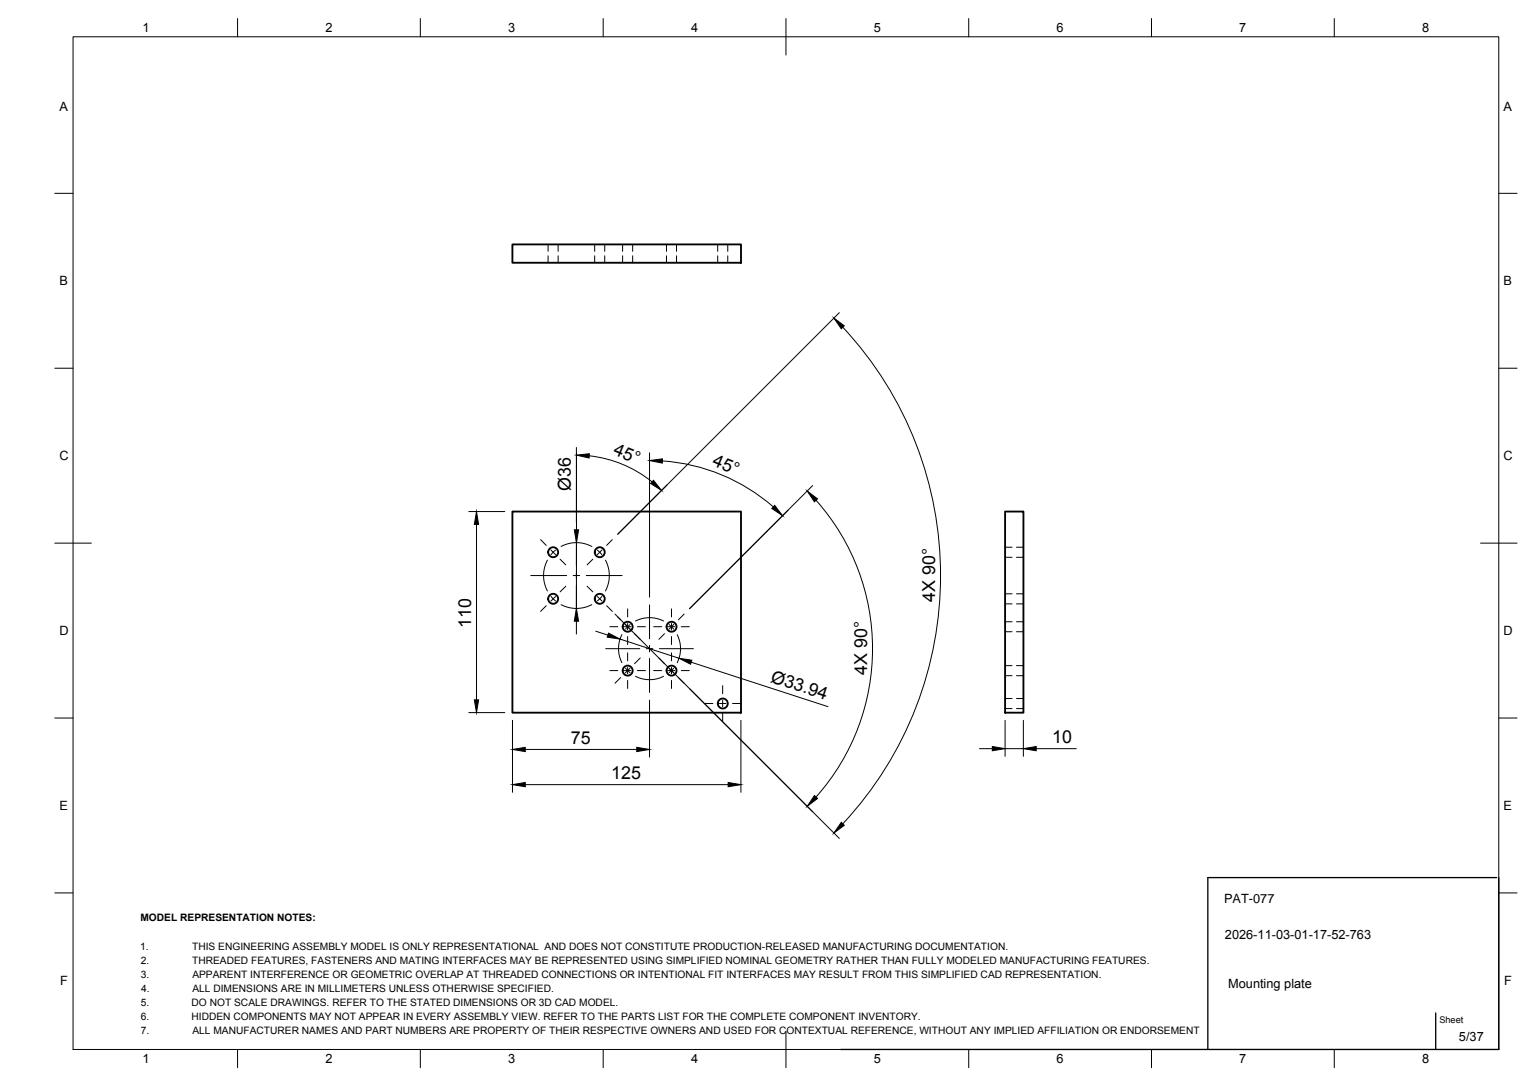
ISO-10303-21;
HEADER;
/* Generated by software containing ST-Developer
 * from STEP Tools, Inc. (www.steptools.com) 
 */

FILE_DESCRIPTION(
/* description */ ('Pallet stop with pneumatic fitting'),
/* implementation_level */ '2;1');

FILE_NAME(
/* name */ 'Mounting plate.step',
/* time_stamp */ '2026-10-27T10:51:41-07:00',
/* author */ (''),
/* organization */ (''),
/* preprocessor_version */ 'ST-DEVELOPER v20.2',
/* originating_system */ 'Autodesk Translation Framework v15.17.0.0',
/* authorisation */ '');

FILE_SCHEMA (('AUTOMOTIVE_DESIGN { 1 0 10303 214 3 1 1 }'));
ENDSEC;

DATA;
#10=MECHANICAL_DESIGN_GEOMETRIC_PRESENTATION_REPRESENTATION('',(#357),#10265);
#293=SHAPE_REPRESENTATION_RELATIONSHIP('SRR','None',#10406,#325);
#325=ADVANCED_BREP_SHAPE_REPRESENTATION('',(#389),#10230);
#357=STYLED_ITEM('',(#10641),#389);
#389=MANIFOLD_SOLID_BREP('Body1',#5045);
#419=FACE_BOUND('',#1064,.T.);
#420=FACE_BOUND('',#1065,.T.);
#421=FACE_BOUND('',#1066,.T.);
#422=FACE_BOUND('',#1067,.T.);
#423=FACE_BOUND('',#1068,.T.);
#424=FACE_BOUND('',#1069,.T.);
#425=FACE_BOUND('',#1070,.T.);
#426=FACE_BOUND('',#1071,.T.);
#427=FACE_BOUND('',#1072,.T.);
#428=FACE_BOUND('',#1074,.T.);
#429=FACE_BOUND('',#1075,.T.);
#430=FACE_BOUND('',#1076,.T.);
#431=FACE_BOUND('',#1077,.T.);
#432=FACE_BOUND('',#1078,.T.);
#433=FACE_BOUND('',#1079,.T.);
#434=FACE_BOUND('',#1080,.T.);
#435=FACE_BOUND('',#1081,.T.);
#436=FACE_BOUND('',#1082,.T.);
#545=PLANE('',#5462);
#546=PLANE('',#5463);
#547=PLANE('',#5464);
#548=PLANE('',#5465);
#549=PLANE('',#5466);
#550=PLANE('',#5467);
#736=FACE_OUTER_BOUND('',#1050,.T.);
#737=FACE_OUTER_BOUND('',#1051,.T.);
#738=FACE_OUTER_BOUND('',#1052,.T.);
#739=FACE_OUTER_BOUND('',#1053,.T.);
#740=FACE_OUTER_BOUND('',#1054,.T.);
#741=FACE_OUTER_BOUND('',#1055,.T.);
#742=FACE_OUTER_BOUND('',#1056,.T.);
#743=FACE_OUTER_BOUND('',#1057,.T.);
#744=FACE_OUTER_BOUND('',#1058,.T.);
#745=FACE_OUTER_BOUND('',#1059,.T.);
#746=FACE_OUTER_BOUND('',#1060,.T.);
#747=FACE_OUTER_BOUND('',#1061,.T.);
#748=FACE_OUTER_BOUND('',#1062,.T.);
#749=FACE_OUTER_BOUND('',#1063,.T.);
#750=FACE_OUTER_BOUND('',#1073,.T.);
#1050=EDGE_LOOP('',(#3410,#3411,#3412,#3413));
#1051=EDGE_LOOP('',(#3414,#3415,#3416,#3417));
#1052=EDGE_LOOP('',(#3418,#3419,#3420,#3421));
#1053=EDGE_LOOP('',(#3422,#3423,#3424,#3425));
#1054=EDGE_LOOP('',(#3426,#3427,#3428,#3429));
#1055=EDGE_LOOP('',(#3430,#3431,#3432,#3433));
#1056=EDGE_LOOP('',(#3434,#3435,#3436,#3437));
#1057=EDGE_LOOP('',(#3438,#3439,#3440,#3441));
#1058=EDGE_LOOP('',(#3442,#3443,#3444,#3445));
#1059=EDGE_LOOP('',(#3446,#3447,#3448,#3449));
#1060=EDGE_LOOP('',(#3450,#3451,#3452,#3453));
#1061=EDGE_LOOP('',(#3454,#3455,#3456,#3457));
#1062=EDGE_LOOP('',(#3458,#3459,#3460,#3461));
#1063=EDGE_LOOP('',(#3462,#3463,#3464,#3465));
#1064=EDGE_LOOP('',(#3466));
#1065=EDGE_LOOP('',(#3467));
#1066=EDGE_LOOP('',(#3468));
#1067=EDGE_LOOP('',(#3469));
#1068=EDGE_LOOP('',(#3470));
#1069=EDGE_LOOP('',(#3471));
#1070=EDGE_LOOP('',(#3472));
#1071=EDGE_LOOP('',(#3473));
#1072=EDGE_LOOP('',(#3474));
#1073=EDGE_LOOP('',(#3475,#3476,#3477,#3478));
#1074=EDGE_LOOP('',(#3479));
#1075=EDGE_LOOP('',(#3480));
#1076=EDGE_LOOP('',(#3481));
#1077=EDGE_LOOP('',(#3482));
#1078=EDGE_LOOP('',(#3483));
#1079=EDGE_LOOP('',(#3484));
#1080=EDGE_LOOP('',(#3485));
#1081=EDGE_LOOP('',(#3486));
#1082=EDGE_LOOP('',(#3487));
#1490=LINE('',#7745,#1825);
#1491=LINE('',#7751,#1826);
#1492=LINE('',#7757,#1827);
#1493=LINE('',#7763,#1828);
#1494=LINE('',#7769,#1829);
#1495=LINE('',#7775,#1830);
#1496=LINE('',#7781,#1831);
#1497=LINE('',#7787,#1832);
#1498=LINE('',#7793,#1833);
#1499=LINE('',#7798,#1834);
#1500=LINE('',#7800,#1835);
#1501=LINE('',#7802,#1836);
#1502=LINE('',#7803,#1837);
#1503=LINE('',#7806,#1838);
#1504=LINE('',#7808,#1839);
#1505=LINE('',#7809,#1840);
#1506=LINE('',#7812,#1841);
#1507=LINE('',#7814,#1842);
#1508=LINE('',#7815,#1843);
#1509=LINE('',#7817,#1844);
#1510=LINE('',#7818,#1845);
#1825=VECTOR('',#6099,0.275);
#1826=VECTOR('',#6106,0.275);
#1827=VECTOR('',#6113,0.275);
#1828=VECTOR('',#6120,0.275);
#1829=VECTOR('',#6127,0.275);
#1830=VECTOR('',#6134,0.275);
#1831=VECTOR('',#6141,0.275);
#1832=VECTOR('',#6148,0.275);
#1833=VECTOR('',#6155,0.275);
#1834=VECTOR('',#6160,1.);
#1835=VECTOR('',#6161,1.);
#1836=VECTOR('',#6162,1.);
#1837=VECTOR('',#6163,1.);
#1838=VECTOR('',#6166,1.);
#1839=VECTOR('',#6167,1.);
#1840=VECTOR('',#6168,1.);
#1841=VECTOR('',#6171,1.);
#1842=VECTOR('',#6172,1.);
#1843=VECTOR('',#6173,1.);
#1844=VECTOR('',#6176,1.);
#1845=VECTOR('',#6177,1.);
#2160=CIRCLE('',#5436,0.275);
#2161=CIRCLE('',#5437,0.275);
#2162=CIRCLE('',#5439,0.275);
#2163=CIRCLE('',#5440,0.275);
#2164=CIRCLE('',#5442,0.275);
#2165=CIRCLE('',#5443,0.275);
#2166=CIRCLE('',#5445,0.275);
#2167=CIRCLE('',#5446,0.275);
#2168=CIRCLE('',#5448,0.275);
#2169=CIRCLE('',#5449,0.275);
#2170=CIRCLE('',#5451,0.275);
#2171=CIRCLE('',#5452,0.275);
#2172=CIRCLE('',#5454,0.275);
#2173=CIRCLE('',#5455,0.275);
#2174=CIRCLE('',#5457,0.275);
#2175=CIRCLE('',#5458,0.275);
#2176=CIRCLE('',#5460,0.275);
#2177=CIRCLE('',#5461,0.275);
#2407=VERTEX_POINT('',#7742);
#2408=VERTEX_POINT('',#7744);
#2409=VERTEX_POINT('',#7748);
#2410=VERTEX_POINT('',#7750);
#2411=VERTEX_POINT('',#7754);
#2412=VERTEX_POINT('',#7756);
#2413=VERTEX_POINT('',#7760);
#2414=VERTEX_POINT('',#7762);
#2415=VERTEX_POINT('',#7766);
#2416=VERTEX_POINT('',#7768);
#2417=VERTEX_POINT('',#7772);
#2418=VERTEX_POINT('',#7774);
#2419=VERTEX_POINT('',#7778);
#2420=VERTEX_POINT('',#7780);
#2421=VERTEX_POINT('',#7784);
#2422=VERTEX_POINT('',#7786);
#2423=VERTEX_POINT('',#7790);
#2424=VERTEX_POINT('',#7792);
#2425=VERTEX_POINT('',#7796);
#2426=VERTEX_POINT('',#7797);
#2427=VERTEX_POINT('',#7799);
#2428=VERTEX_POINT('',#7801);
#2429=VERTEX_POINT('',#7805);
#2430=VERTEX_POINT('',#7807);
#2431=VERTEX_POINT('',#7811);
#2432=VERTEX_POINT('',#7813);
#2804=EDGE_CURVE('',#2407,#2407,#2160,.T.);
#2805=EDGE_CURVE('',#2407,#2408,#1490,.T.);
#2806=EDGE_CURVE('',#2408,#2408,#2161,.T.);
#2807=EDGE_CURVE('',#2409,#2409,#2162,.T.);
#2808=EDGE_CURVE('',#2409,#2410,#1491,.T.);
#2809=EDGE_CURVE('',#2410,#2410,#2163,.T.);
#2810=EDGE_CURVE('',#2411,#2411,#2164,.T.);
#2811=EDGE_CURVE('',#2411,#2412,#1492,.T.);
#2812=EDGE_CURVE('',#2412,#2412,#2165,.T.);
#2813=EDGE_CURVE('',#2413,#2413,#2166,.T.);
#2814=EDGE_CURVE('',#2413,#2414,#1493,.T.);
#2815=EDGE_CURVE('',#2414,#2414,#2167,.T.);
#2816=EDGE_CURVE('',#2415,#2415,#2168,.T.);
#2817=EDGE_CURVE('',#2415,#2416,#1494,.T.);
#2818=EDGE_CURVE('',#2416,#2416,#2169,.T.);
#2819=EDGE_CURVE('',#2417,#2417,#2170,.T.);
#2820=EDGE_CURVE('',#2417,#2418,#1495,.T.);
#2821=EDGE_CURVE('',#2418,#2418,#2171,.T.);
#2822=EDGE_CURVE('',#2419,#2419,#2172,.T.);
#2823=EDGE_CURVE('',#2419,#2420,#1496,.T.);
#2824=EDGE_CURVE('',#2420,#2420,#2173,.T.);
#2825=EDGE_CURVE('',#2421,#2421,#2174,.T.);
#2826=EDGE_CURVE('',#2421,#2422,#1497,.T.);
#2827=EDGE_CURVE('',#2422,#2422,#2175,.T.);
#2828=EDGE_CURVE('',#2423,#2423,#2176,.T.);
#2829=EDGE_CURVE('',#2423,#2424,#1498,.T.);
#2830=EDGE_CURVE('',#2424,#2424,#2177,.T.);
#2831=EDGE_CURVE('',#2425,#2426,#1499,.T.);
#2832=EDGE_CURVE('',#2426,#2427,#1500,.T.);
#2833=EDGE_CURVE('',#2428,#2427,#1501,.T.);
#2834=EDGE_CURVE('',#2425,#2428,#1502,.T.);
#2835=EDGE_CURVE('',#2429,#2425,#1503,.T.);
#2836=EDGE_CURVE('',#2430,#2428,#1504,.T.);
#2837=EDGE_CURVE('',#2429,#2430,#1505,.T.);
#2838=EDGE_CURVE('',#2431,#2429,#1506,.T.);
#2839=EDGE_CURVE('',#2432,#2430,#1507,.T.);
#2840=EDGE_CURVE('',#2431,#2432,#1508,.T.);
#2841=EDGE_CURVE('',#2426,#2431,#1509,.T.);
#2842=EDGE_CURVE('',#2427,#2432,#1510,.T.);
#3410=ORIENTED_EDGE('',*,*,#2804,.F.);
#3411=ORIENTED_EDGE('',*,*,#2805,.T.);
#3412=ORIENTED_EDGE('',*,*,#2806,.F.);
#3413=ORIENTED_EDGE('',*,*,#2805,.F.);
#3414=ORIENTED_EDGE('',*,*,#2807,.F.);
#3415=ORIENTED_EDGE('',*,*,#2808,.T.);
#3416=ORIENTED_EDGE('',*,*,#2809,.F.);
#3417=ORIENTED_EDGE('',*,*,#2808,.F.);
#3418=ORIENTED_EDGE('',*,*,#2810,.F.);
#3419=ORIENTED_EDGE('',*,*,#2811,.T.);
#3420=ORIENTED_EDGE('',*,*,#2812,.F.);
#3421=ORIENTED_EDGE('',*,*,#2811,.F.);
#3422=ORIENTED_EDGE('',*,*,#2813,.F.);
#3423=ORIENTED_EDGE('',*,*,#2814,.T.);
#3424=ORIENTED_EDGE('',*,*,#2815,.F.);
#3425=ORIENTED_EDGE('',*,*,#2814,.F.);
#3426=ORIENTED_EDGE('',*,*,#2816,.F.);
#3427=ORIENTED_EDGE('',*,*,#2817,.T.);
#3428=ORIENTED_EDGE('',*,*,#2818,.F.);
#3429=ORIENTED_EDGE('',*,*,#2817,.F.);
#3430=ORIENTED_EDGE('',*,*,#2819,.F.);
#3431=ORIENTED_EDGE('',*,*,#2820,.T.);
#3432=ORIENTED_EDGE('',*,*,#2821,.F.);
#3433=ORIENTED_EDGE('',*,*,#2820,.F.);
#3434=ORIENTED_EDGE('',*,*,#2822,.F.);
#3435=ORIENTED_EDGE('',*,*,#2823,.T.);
#3436=ORIENTED_EDGE('',*,*,#2824,.F.);
#3437=ORIENTED_EDGE('',*,*,#2823,.F.);
#3438=ORIENTED_EDGE('',*,*,#2825,.F.);
#3439=ORIENTED_EDGE('',*,*,#2826,.T.);
#3440=ORIENTED_EDGE('',*,*,#2827,.F.);
#3441=ORIENTED_EDGE('',*,*,#2826,.F.);
#3442=ORIENTED_EDGE('',*,*,#2828,.F.);
#3443=ORIENTED_EDGE('',*,*,#2829,.T.);
#3444=ORIENTED_EDGE('',*,*,#2830,.F.);
#3445=ORIENTED_EDGE('',*,*,#2829,.F.);
#3446=ORIENTED_EDGE('',*,*,#2831,.T.);
#3447=ORIENTED_EDGE('',*,*,#2832,.T.);
#3448=ORIENTED_EDGE('',*,*,#2833,.F.);
#3449=ORIENTED_EDGE('',*,*,#2834,.F.);
#3450=ORIENTED_EDGE('',*,*,#2835,.T.);
#3451=ORIENTED_EDGE('',*,*,#2834,.T.);
#3452=ORIENTED_EDGE('',*,*,#2836,.F.);
#3453=ORIENTED_EDGE('',*,*,#2837,.F.);
#3454=ORIENTED_EDGE('',*,*,#2838,.T.);
#3455=ORIENTED_EDGE('',*,*,#2837,.T.);
#3456=ORIENTED_EDGE('',*,*,#2839,.F.);
#3457=ORIENTED_EDGE('',*,*,#2840,.F.);
#3458=ORIENTED_EDGE('',*,*,#2841,.T.);
#3459=ORIENTED_EDGE('',*,*,#2840,.T.);
#3460=ORIENTED_EDGE('',*,*,#2842,.F.);
#3461=ORIENTED_EDGE('',*,*,#2832,.F.);
#3462=ORIENTED_EDGE('',*,*,#2842,.T.);
#3463=ORIENTED_EDGE('',*,*,#2839,.T.);
#3464=ORIENTED_EDGE('',*,*,#2836,.T.);
#3465=ORIENTED_EDGE('',*,*,#2833,.T.);
#3466=ORIENTED_EDGE('',*,*,#2830,.T.);
#3467=ORIENTED_EDGE('',*,*,#2827,.T.);
#3468=ORIENTED_EDGE('',*,*,#2824,.T.);
#3469=ORIENTED_EDGE('',*,*,#2821,.T.);
#3470=ORIENTED_EDGE('',*,*,#2818,.T.);
#3471=ORIENTED_EDGE('',*,*,#2815,.T.);
#3472=ORIENTED_EDGE('',*,*,#2812,.T.);
#3473=ORIENTED_EDGE('',*,*,#2809,.T.);
#3474=ORIENTED_EDGE('',*,*,#2806,.T.);
#3475=ORIENTED_EDGE('',*,*,#2841,.F.);
#3476=ORIENTED_EDGE('',*,*,#2831,.F.);
#3477=ORIENTED_EDGE('',*,*,#2835,.F.);
#3478=ORIENTED_EDGE('',*,*,#2838,.F.);
#3479=ORIENTED_EDGE('',*,*,#2828,.T.);
#3480=ORIENTED_EDGE('',*,*,#2825,.T.);
#3481=ORIENTED_EDGE('',*,*,#2822,.T.);
#3482=ORIENTED_EDGE('',*,*,#2819,.T.);
#3483=ORIENTED_EDGE('',*,*,#2816,.T.);
#3484=ORIENTED_EDGE('',*,*,#2813,.T.);
#3485=ORIENTED_EDGE('',*,*,#2810,.T.);
#3486=ORIENTED_EDGE('',*,*,#2807,.T.);
#3487=ORIENTED_EDGE('',*,*,#2804,.T.);
#4622=CYLINDRICAL_SURFACE('',#5435,0.275);
#4623=CYLINDRICAL_SURFACE('',#5438,0.275);
#4624=CYLINDRICAL_SURFACE('',#5441,0.275);
#4625=CYLINDRICAL_SURFACE('',#5444,0.275);
#4626=CYLINDRICAL_SURFACE('',#5447,0.275);
#4627=CYLINDRICAL_SURFACE('',#5450,0.275);
#4628=CYLINDRICAL_SURFACE('',#5453,0.275);
#4629=CYLINDRICAL_SURFACE('',#5456,0.275);
#4630=CYLINDRICAL_SURFACE('',#5459,0.275);
#4731=ADVANCED_FACE('',(#736),#4622,.F.);
#4732=ADVANCED_FACE('',(#737),#4623,.F.);
#4733=ADVANCED_FACE('',(#738),#4624,.F.);
#4734=ADVANCED_FACE('',(#739),#4625,.F.);
#4735=ADVANCED_FACE('',(#740),#4626,.F.);
#4736=ADVANCED_FACE('',(#741),#4627,.F.);
#4737=ADVANCED_FACE('',(#742),#4628,.F.);
#4738=ADVANCED_FACE('',(#743),#4629,.F.);
#4739=ADVANCED_FACE('',(#744),#4630,.F.);
#4740=ADVANCED_FACE('',(#745),#545,.T.);
#4741=ADVANCED_FACE('',(#746),#546,.T.);
#4742=ADVANCED_FACE('',(#747),#547,.T.);
#4743=ADVANCED_FACE('',(#748),#548,.T.);
#4744=ADVANCED_FACE('',(#749,#419,#420,#421,#422,#423,#424,#425,#426,#427),
#549,.T.);
#4745=ADVANCED_FACE('',(#750,#428,#429,#430,#431,#432,#433,#434,#435,#436),
#550,.F.);
#5045=CLOSED_SHELL('',(#4731,#4732,#4733,#4734,#4735,#4736,#4737,#4738,
#4739,#4740,#4741,#4742,#4743,#4744,#4745));
#5434=AXIS2_PLACEMENT_3D('',#7740,#6093,#6094);
#5435=AXIS2_PLACEMENT_3D('',#7741,#6095,#6096);
#5436=AXIS2_PLACEMENT_3D('',#7743,#6097,#6098);
#5437=AXIS2_PLACEMENT_3D('',#7746,#6100,#6101);
#5438=AXIS2_PLACEMENT_3D('',#7747,#6102,#6103);
#5439=AXIS2_PLACEMENT_3D('',#7749,#6104,#6105);
#5440=AXIS2_PLACEMENT_3D('',#7752,#6107,#6108);
#5441=AXIS2_PLACEMENT_3D('',#7753,#6109,#6110);
#5442=AXIS2_PLACEMENT_3D('',#7755,#6111,#6112);
#5443=AXIS2_PLACEMENT_3D('',#7758,#6114,#6115);
#5444=AXIS2_PLACEMENT_3D('',#7759,#6116,#6117);
#5445=AXIS2_PLACEMENT_3D('',#7761,#6118,#6119);
#5446=AXIS2_PLACEMENT_3D('',#7764,#6121,#6122);
#5447=AXIS2_PLACEMENT_3D('',#7765,#6123,#6124);
#5448=AXIS2_PLACEMENT_3D('',#7767,#6125,#6126);
#5449=AXIS2_PLACEMENT_3D('',#7770,#6128,#6129);
#5450=AXIS2_PLACEMENT_3D('',#7771,#6130,#6131);
#5451=AXIS2_PLACEMENT_3D('',#7773,#6132,#6133);
#5452=AXIS2_PLACEMENT_3D('',#7776,#6135,#6136);
#5453=AXIS2_PLACEMENT_3D('',#7777,#6137,#6138);
#5454=AXIS2_PLACEMENT_3D('',#7779,#6139,#6140);
#5455=AXIS2_PLACEMENT_3D('',#7782,#6142,#6143);
#5456=AXIS2_PLACEMENT_3D('',#7783,#6144,#6145);
#5457=AXIS2_PLACEMENT_3D('',#7785,#6146,#6147);
#5458=AXIS2_PLACEMENT_3D('',#7788,#6149,#6150);
#5459=AXIS2_PLACEMENT_3D('',#7789,#6151,#6152);
#5460=AXIS2_PLACEMENT_3D('',#7791,#6153,#6154);
#5461=AXIS2_PLACEMENT_3D('',#7794,#6156,#6157);
#5462=AXIS2_PLACEMENT_3D('',#7795,#6158,#6159);
#5463=AXIS2_PLACEMENT_3D('',#7804,#6164,#6165);
#5464=AXIS2_PLACEMENT_3D('',#7810,#6169,#6170);
#5465=AXIS2_PLACEMENT_3D('',#7816,#6174,#6175);
#5466=AXIS2_PLACEMENT_3D('',#7819,#6178,#6179);
#5467=AXIS2_PLACEMENT_3D('',#7820,#6180,#6181);
#6093=DIRECTION('axis',(0.,0.,1.));
#6094=DIRECTION('refdir',(1.,0.,0.));
#6095=DIRECTION('center_axis',(0.,0.,1.));
#6096=DIRECTION('ref_axis',(1.,0.,0.));
#6097=DIRECTION('center_axis',(0.,0.,1.));
#6098=DIRECTION('ref_axis',(1.,0.,0.));
#6099=DIRECTION('',(0.,0.,1.));
#6100=DIRECTION('center_axis',(0.,0.,-1.));
#6101=DIRECTION('ref_axis',(1.,0.,0.));
#6102=DIRECTION('center_axis',(0.,0.,1.));
#6103=DIRECTION('ref_axis',(1.,0.,0.));
#6104=DIRECTION('center_axis',(0.,0.,1.));
#6105=DIRECTION('ref_axis',(1.,0.,0.));
#6106=DIRECTION('',(0.,0.,1.));
#6107=DIRECTION('center_axis',(0.,0.,-1.));
#6108=DIRECTION('ref_axis',(1.,0.,0.));
#6109=DIRECTION('center_axis',(0.,0.,1.));
#6110=DIRECTION('ref_axis',(1.,0.,0.));
#6111=DIRECTION('center_axis',(0.,0.,1.));
#6112=DIRECTION('ref_axis',(1.,0.,0.));
#6113=DIRECTION('',(0.,0.,1.));
#6114=DIRECTION('center_axis',(0.,0.,-1.));
#6115=DIRECTION('ref_axis',(1.,0.,0.));
#6116=DIRECTION('center_axis',(0.,0.,1.));
#6117=DIRECTION('ref_axis',(1.,0.,0.));
#6118=DIRECTION('center_axis',(0.,0.,1.));
#6119=DIRECTION('ref_axis',(1.,0.,0.));
#6120=DIRECTION('',(0.,0.,1.));
#6121=DIRECTION('center_axis',(0.,0.,-1.));
#6122=DIRECTION('ref_axis',(1.,0.,0.));
#6123=DIRECTION('center_axis',(0.,0.,1.));
#6124=DIRECTION('ref_axis',(1.,0.,0.));
#6125=DIRECTION('center_axis',(0.,0.,1.));
#6126=DIRECTION('ref_axis',(1.,0.,0.));
#6127=DIRECTION('',(0.,0.,1.));
#6128=DIRECTION('center_axis',(0.,0.,-1.));
#6129=DIRECTION('ref_axis',(1.,0.,0.));
#6130=DIRECTION('center_axis',(0.,0.,1.));
#6131=DIRECTION('ref_axis',(1.,0.,0.));
#6132=DIRECTION('center_axis',(0.,0.,1.));
#6133=DIRECTION('ref_axis',(1.,0.,0.));
#6134=DIRECTION('',(0.,0.,1.));
#6135=DIRECTION('center_axis',(0.,0.,-1.));
#6136=DIRECTION('ref_axis',(1.,0.,0.));
#6137=DIRECTION('center_axis',(0.,0.,1.));
#6138=DIRECTION('ref_axis',(1.,0.,0.));
#6139=DIRECTION('center_axis',(0.,0.,1.));
#6140=DIRECTION('ref_axis',(1.,0.,0.));
#6141=DIRECTION('',(0.,0.,1.));
#6142=DIRECTION('center_axis',(0.,0.,-1.));
#6143=DIRECTION('ref_axis',(1.,0.,0.));
#6144=DIRECTION('center_axis',(0.,0.,1.));
#6145=DIRECTION('ref_axis',(1.,0.,0.));
#6146=DIRECTION('center_axis',(0.,0.,1.));
#6147=DIRECTION('ref_axis',(1.,0.,0.));
#6148=DIRECTION('',(0.,0.,1.));
#6149=DIRECTION('center_axis',(0.,0.,-1.));
#6150=DIRECTION('ref_axis',(1.,0.,0.));
#6151=DIRECTION('center_axis',(0.,0.,1.));
#6152=DIRECTION('ref_axis',(1.,0.,0.));
#6153=DIRECTION('center_axis',(0.,0.,1.));
#6154=DIRECTION('ref_axis',(1.,0.,0.));
#6155=DIRECTION('',(0.,0.,1.));
#6156=DIRECTION('center_axis',(0.,0.,-1.));
#6157=DIRECTION('ref_axis',(1.,0.,0.));
#6158=DIRECTION('center_axis',(0.,1.,0.));
#6159=DIRECTION('ref_axis',(-1.,0.,0.));
#6160=DIRECTION('',(-1.,0.,0.));
#6161=DIRECTION('',(0.,0.,1.));
#6162=DIRECTION('',(-1.,0.,0.));
#6163=DIRECTION('',(0.,0.,1.));
#6164=DIRECTION('center_axis',(1.,0.,0.));
#6165=DIRECTION('ref_axis',(0.,1.,0.));
#6166=DIRECTION('',(0.,1.,0.));
#6167=DIRECTION('',(0.,1.,0.));
#6168=DIRECTION('',(0.,0.,1.));
#6169=DIRECTION('center_axis',(0.,-1.,0.));
#6170=DIRECTION('ref_axis',(1.,0.,0.));
#6171=DIRECTION('',(1.,0.,0.));
#6172=DIRECTION('',(1.,0.,0.));
#6173=DIRECTION('',(0.,0.,1.));
#6174=DIRECTION('center_axis',(-1.,0.,0.));
#6175=DIRECTION('ref_axis',(0.,-1.,0.));
#6176=DIRECTION('',(0.,-1.,0.));
#6177=DIRECTION('',(0.,-1.,0.));
#6178=DIRECTION('center_axis',(0.,0.,1.));
#6179=DIRECTION('ref_axis',(1.,0.,0.));
#6180=DIRECTION('center_axis',(0.,0.,1.));
#6181=DIRECTION('ref_axis',(1.,0.,0.));
#7740=CARTESIAN_POINT('',(0.,0.,0.));
#7741=CARTESIAN_POINT('Origin',(2.72720779386421,2.72720779386421,-1.1));
#7742=CARTESIAN_POINT('',(2.45220779386421,2.72720779386421,-1.));
#7743=CARTESIAN_POINT('Origin',(2.72720779386421,2.72720779386421,-1.));
#7744=CARTESIAN_POINT('',(2.45220779386421,2.72720779386421,0.));
#7745=CARTESIAN_POINT('',(2.45220779386421,2.72720779386421,-1.1));
#7746=CARTESIAN_POINT('Origin',(2.72720779386421,2.72720779386421,0.));
#7747=CARTESIAN_POINT('Origin',(2.72720779386421,5.27279220613579,-1.1));
#7748=CARTESIAN_POINT('',(2.45220779386421,5.27279220613579,-1.));
#7749=CARTESIAN_POINT('Origin',(2.72720779386421,5.27279220613579,-1.));
#7750=CARTESIAN_POINT('',(2.45220779386421,5.27279220613579,0.));
#7751=CARTESIAN_POINT('',(2.45220779386421,5.27279220613579,-1.1));
#7752=CARTESIAN_POINT('Origin',(2.72720779386421,5.27279220613579,0.));
#7753=CARTESIAN_POINT('Origin',(5.27279220613579,5.27279220613579,-1.1));
#7754=CARTESIAN_POINT('',(4.99779220613579,5.27279220613579,-1.));
#7755=CARTESIAN_POINT('Origin',(5.27279220613579,5.27279220613579,-1.));
#7756=CARTESIAN_POINT('',(4.99779220613579,5.27279220613579,0.));
#7757=CARTESIAN_POINT('',(4.99779220613579,5.27279220613579,-1.1));
#7758=CARTESIAN_POINT('Origin',(5.27279220613579,5.27279220613579,0.));
#7759=CARTESIAN_POINT('Origin',(5.27279220613578,2.72720779386421,-1.1));
#7760=CARTESIAN_POINT('',(4.99779220613578,2.72720779386421,-1.));
#7761=CARTESIAN_POINT('Origin',(5.27279220613578,2.72720779386421,-1.));
#7762=CARTESIAN_POINT('',(4.99779220613578,2.72720779386421,0.));
#7763=CARTESIAN_POINT('',(4.99779220613578,2.72720779386421,-1.1));
#7764=CARTESIAN_POINT('Origin',(5.27279220613578,2.72720779386421,0.));
#7765=CARTESIAN_POINT('Origin',(-4.,-3.,-1.1));
#7766=CARTESIAN_POINT('',(-4.275,-3.,-1.));
#7767=CARTESIAN_POINT('Origin',(-4.,-3.,-1.));
#7768=CARTESIAN_POINT('',(-4.275,-3.,0.));
#7769=CARTESIAN_POINT('',(-4.275,-3.,-1.1));
#7770=CARTESIAN_POINT('Origin',(-4.,-3.,0.));
#7771=CARTESIAN_POINT('Origin',(1.2,-1.2,-1.1));
#7772=CARTESIAN_POINT('',(0.925,-1.2,-1.));
#7773=CARTESIAN_POINT('Origin',(1.2,-1.2,-1.));
#7774=CARTESIAN_POINT('',(0.925,-1.2,0.));
#7775=CARTESIAN_POINT('',(0.925,-1.2,-1.1));
#7776=CARTESIAN_POINT('Origin',(1.2,-1.2,0.));
#7777=CARTESIAN_POINT('Origin',(-1.2,1.2,-1.1));
#7778=CARTESIAN_POINT('',(-1.475,1.2,-1.));
#7779=CARTESIAN_POINT('Origin',(-1.2,1.2,-1.));
#7780=CARTESIAN_POINT('',(-1.475,1.2,0.));
#7781=CARTESIAN_POINT('',(-1.475,1.2,-1.1));
#7782=CARTESIAN_POINT('Origin',(-1.2,1.2,0.));
#7783=CARTESIAN_POINT('Origin',(-1.2,-1.2,-1.1));
#7784=CARTESIAN_POINT('',(-1.475,-1.2,-1.));
#7785=CARTESIAN_POINT('Origin',(-1.2,-1.2,-1.));
#7786=CARTESIAN_POINT('',(-1.475,-1.2,0.));
#7787=CARTESIAN_POINT('',(-1.475,-1.2,-1.1));
#7788=CARTESIAN_POINT('Origin',(-1.2,-1.2,0.));
#7789=CARTESIAN_POINT('Origin',(1.2,1.2,-1.1));
#7790=CARTESIAN_POINT('',(0.925,1.2,-1.));
#7791=CARTESIAN_POINT('Origin',(1.2,1.2,-1.));
#7792=CARTESIAN_POINT('',(0.925,1.2,0.));
#7793=CARTESIAN_POINT('',(0.925,1.2,-1.1));
#7794=CARTESIAN_POINT('Origin',(1.2,1.2,0.));
#7795=CARTESIAN_POINT('Origin',(7.5,7.5,-1.));
#7796=CARTESIAN_POINT('',(7.5,7.5,-1.));
#7797=CARTESIAN_POINT('',(-5.,7.5,-1.));
#7798=CARTESIAN_POINT('',(7.5,7.5,-1.));
#7799=CARTESIAN_POINT('',(-5.,7.5,0.));
#7800=CARTESIAN_POINT('',(-5.,7.5,-1.));
#7801=CARTESIAN_POINT('',(7.5,7.5,0.));
#7802=CARTESIAN_POINT('',(7.5,7.5,0.));
#7803=CARTESIAN_POINT('',(7.5,7.5,-1.));
#7804=CARTESIAN_POINT('Origin',(7.5,-3.5,-1.));
#7805=CARTESIAN_POINT('',(7.5,-3.5,-1.));
#7806=CARTESIAN_POINT('',(7.5,-3.5,-1.));
#7807=CARTESIAN_POINT('',(7.5,-3.5,0.));
#7808=CARTESIAN_POINT('',(7.5,-3.5,0.));
#7809=CARTESIAN_POINT('',(7.5,-3.5,-1.));
#7810=CARTESIAN_POINT('Origin',(-5.,-3.5,-1.));
#7811=CARTESIAN_POINT('',(-5.,-3.5,-1.));
#7812=CARTESIAN_POINT('',(-5.,-3.5,-1.));
#7813=CARTESIAN_POINT('',(-5.,-3.5,0.));
#7814=CARTESIAN_POINT('',(-5.,-3.5,0.));
#7815=CARTESIAN_POINT('',(-5.,-3.5,-1.));
#7816=CARTESIAN_POINT('Origin',(-5.,7.5,-1.));
#7817=CARTESIAN_POINT('',(-5.,7.5,-1.));
#7818=CARTESIAN_POINT('',(-5.,7.5,0.));
#7819=CARTESIAN_POINT('Origin',(1.25,2.,0.));
#7820=CARTESIAN_POINT('Origin',(1.25,2.,-1.));
#10192=UNCERTAINTY_MEASURE_WITH_UNIT(LENGTH_MEASURE(0.001),#10266,
'DISTANCE_ACCURACY_VALUE',
'Maximum model space distance between geometric entities at asserted c
onnectivities');
#10227=UNCERTAINTY_MEASURE_WITH_UNIT(LENGTH_MEASURE(0.001),#10266,
'DISTANCE_ACCURACY_VALUE',
'Maximum model space distance between geometric entities at asserted c
onnectivities');
#10230=(
GEOMETRIC_REPRESENTATION_CONTEXT(3)
GLOBAL_UNCERTAINTY_ASSIGNED_CONTEXT((#10192))
GLOBAL_UNIT_ASSIGNED_CONTEXT((#10266,#10268,#10269))
REPRESENTATION_CONTEXT('','3D')
);
#10265=(
GEOMETRIC_REPRESENTATION_CONTEXT(3)
GLOBAL_UNCERTAINTY_ASSIGNED_CONTEXT((#10227))
GLOBAL_UNIT_ASSIGNED_CONTEXT((#10266,#10268,#10269))
REPRESENTATION_CONTEXT('','3D')
);
#10266=(
LENGTH_UNIT()
NAMED_UNIT(*)
SI_UNIT(.CENTI.,.METRE.)
);
#10268=(
NAMED_UNIT(*)
PLANE_ANGLE_UNIT()
SI_UNIT($,.RADIAN.)
);
#10269=(
NAMED_UNIT(*)
SI_UNIT($,.STERADIAN.)
SOLID_ANGLE_UNIT()
);
#10272=SHAPE_DEFINITION_REPRESENTATION(#10309,#10406);
#10309=PRODUCT_DEFINITION_SHAPE('',$,#10444);
#10406=SHAPE_REPRESENTATION('',(#5434),#10230);
#10441=PRODUCT_DEFINITION_CONTEXT('part definition',#10554,'design');
#10444=PRODUCT_DEFINITION('Mounting plate','Mounting plate',#10481,#10441);
#10481=PRODUCT_DEFINITION_FORMATION('',$,#10558);
#10554=APPLICATION_CONTEXT(
'Core Data for Automotive Mechanical Design Process');
#10555=PRODUCT_CONTEXT('part definition',#10554,'mechanical');
#10558=PRODUCT('Mounting plate','Mounting plate','Mounting plate',(#10555));
#10635=COLOUR_RGB('Light Blue',0.38,0.62,0.78);
#10636=FILL_AREA_STYLE_COLOUR('',#10635);
#10637=FILL_AREA_STYLE('',(#10636));
#10638=SURFACE_STYLE_FILL_AREA(#10637);
#10639=SURFACE_SIDE_STYLE('',(#10638));
#10640=SURFACE_STYLE_USAGE(.BOTH.,#10639);
#10641=PRESENTATION_STYLE_ASSIGNMENT((#10640));
ENDSEC;
END-ISO-10303-21;
